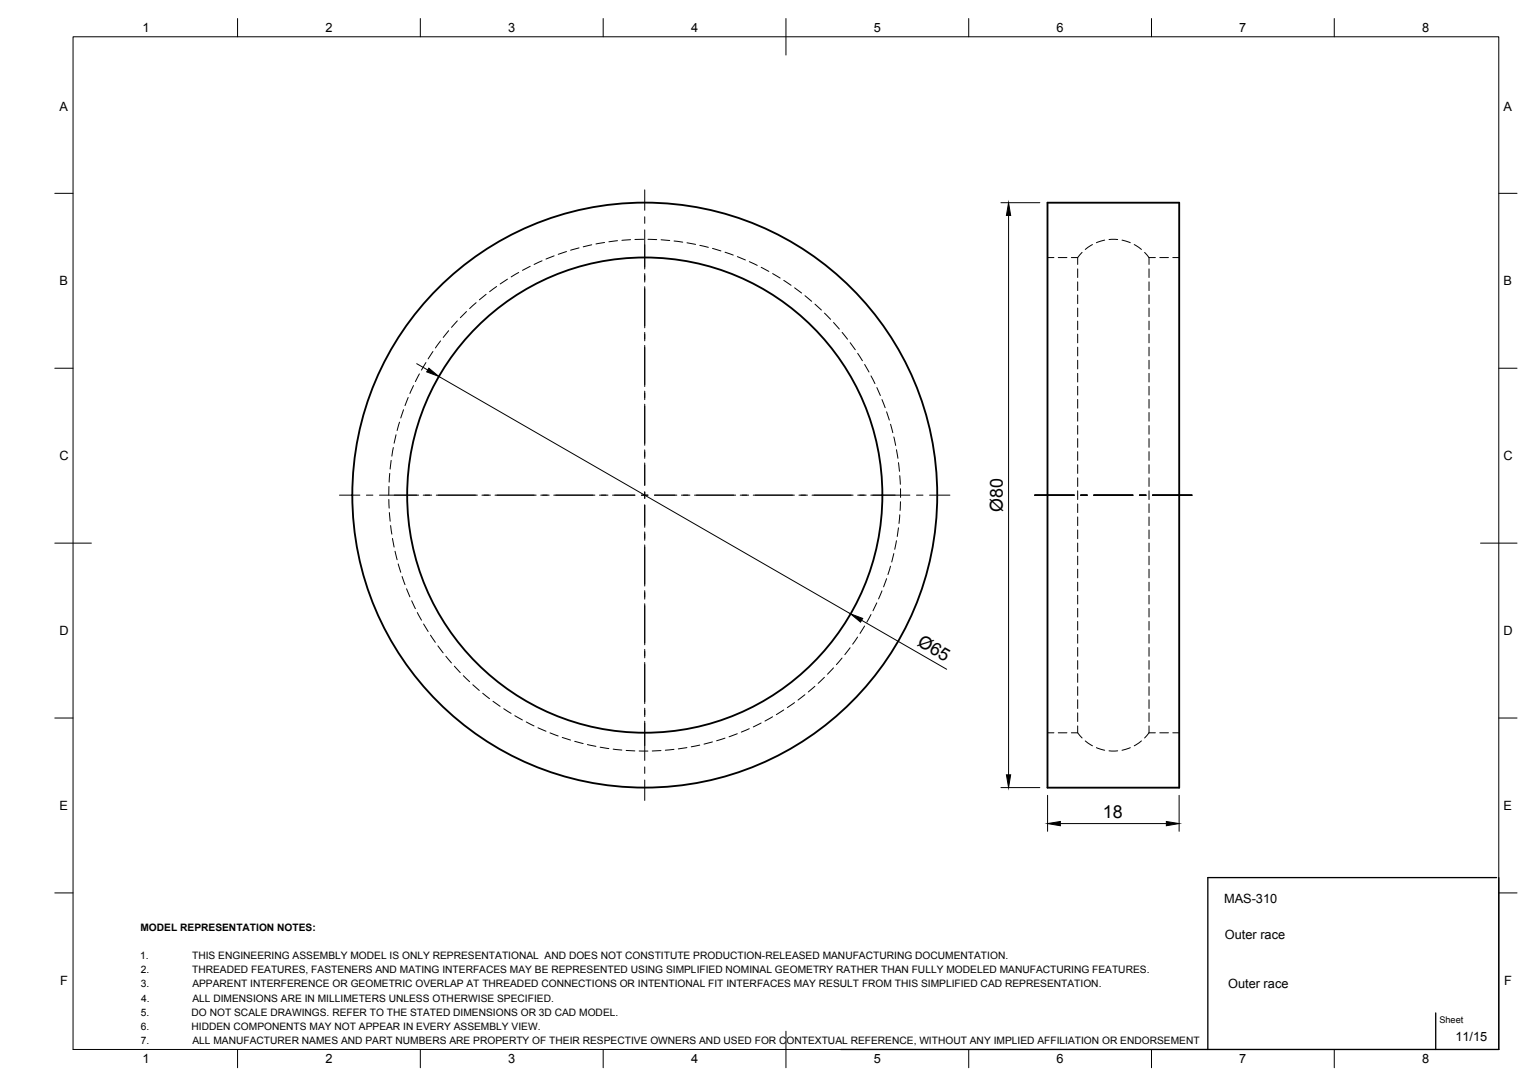
ISO-10303-21;
HEADER;
/* Generated by software containing ST-Developer
 * from STEP Tools, Inc. (www.steptools.com) 
 */

FILE_DESCRIPTION(
/* description */ ('Independent30mm screw-fed quill/spindle unit with16mm straight tool s
ocket, radial set screw, native reusable open ball bearings, retained 
inner/outer race stacks, keyed quill guide and M12x1.75 fine feed. Ext
ernal moving drive and tool not included. Ideal cage orbital links; in
dividual ball spin, force and preload not simulated. No drilling capac
ity, runout, speed, torque, load, life or machine safety rating.'),
/* implementation_level */ '2;1');

FILE_NAME(
/* name */ 'Outer race.step',
/* time_stamp */ '2026-11-08T18:59:42-08:00',
/* author */ (''),
/* organization */ (''),
/* preprocessor_version */ 'ST-DEVELOPER v20.2',
/* originating_system */ 'Autodesk Translation Framework v15.17.0.0',
/* authorisation */ '');

FILE_SCHEMA (('AUTOMOTIVE_DESIGN { 1 0 10303 214 3 1 1 }'));
ENDSEC;

DATA;
#10=MECHANICAL_DESIGN_GEOMETRIC_PRESENTATION_REPRESENTATION('',(#1605),#63898);
#237=TOROIDAL_SURFACE('',#16635,29.,6.);
#1569=SHAPE_REPRESENTATION_RELATIONSHIP('SRR','None',#64008,#1587);
#1587=ADVANCED_BREP_SHAPE_REPRESENTATION('',(#1623),#63893);
#1605=STYLED_ITEM('',(#64103),#1623);
#1623=MANIFOLD_SOLID_BREP('Body1',#15491);
#1708=FACE_BOUND('',#4335,.T.);
#1709=FACE_BOUND('',#4337,.T.);
#2338=CYLINDRICAL_SURFACE('',#16639,32.5);
#2339=CYLINDRICAL_SURFACE('',#16641,32.5);
#2340=CYLINDRICAL_SURFACE('',#16643,40.);
#2577=CIRCLE('',#16636,32.5);
#2578=CIRCLE('',#16637,6.);
#2579=CIRCLE('',#16638,32.5);
#2580=CIRCLE('',#16640,32.5);
#2581=CIRCLE('',#16642,32.5);
#2582=CIRCLE('',#16644,40.);
#2583=CIRCLE('',#16645,40.);
#3412=FACE_OUTER_BOUND('',#4330,.T.);
#3413=FACE_OUTER_BOUND('',#4331,.T.);
#3414=FACE_OUTER_BOUND('',#4332,.T.);
#3415=FACE_OUTER_BOUND('',#4333,.T.);
#3416=FACE_OUTER_BOUND('',#4334,.T.);
#3417=FACE_OUTER_BOUND('',#4336,.T.);
#4330=EDGE_LOOP('',(#14010,#14011,#14012,#14013));
#4331=EDGE_LOOP('',(#14014,#14015,#14016,#14017));
#4332=EDGE_LOOP('',(#14018,#14019,#14020,#14021));
#4333=EDGE_LOOP('',(#14022,#14023,#14024,#14025));
#4334=EDGE_LOOP('',(#14026));
#4335=EDGE_LOOP('',(#14027));
#4336=EDGE_LOOP('',(#14028));
#4337=EDGE_LOOP('',(#14029));
#5127=LINE('',#60412,#5890);
#5128=LINE('',#60415,#5891);
#5129=LINE('',#60421,#5892);
#5890=VECTOR('',#19455,32.5);
#5891=VECTOR('',#19458,32.5);
#5892=VECTOR('',#19465,40.);
#7336=VERTEX_POINT('',#60404);
#7337=VERTEX_POINT('',#60406);
#7338=VERTEX_POINT('',#60410);
#7339=VERTEX_POINT('',#60414);
#7340=VERTEX_POINT('',#60418);
#7341=VERTEX_POINT('',#60420);
#9594=EDGE_CURVE('',#7336,#7336,#2577,.T.);
#9595=EDGE_CURVE('',#7336,#7337,#2578,.T.);
#9596=EDGE_CURVE('',#7337,#7337,#2579,.T.);
#9597=EDGE_CURVE('',#7338,#7338,#2580,.T.);
#9598=EDGE_CURVE('',#7338,#7337,#5127,.T.);
#9599=EDGE_CURVE('',#7336,#7339,#5128,.T.);
#9600=EDGE_CURVE('',#7339,#7339,#2581,.T.);
#9601=EDGE_CURVE('',#7340,#7340,#2582,.T.);
#9602=EDGE_CURVE('',#7340,#7341,#5129,.T.);
#9603=EDGE_CURVE('',#7341,#7341,#2583,.T.);
#14010=ORIENTED_EDGE('',*,*,#9594,.F.);
#14011=ORIENTED_EDGE('',*,*,#9595,.T.);
#14012=ORIENTED_EDGE('',*,*,#9596,.F.);
#14013=ORIENTED_EDGE('',*,*,#9595,.F.);
#14014=ORIENTED_EDGE('',*,*,#9597,.F.);
#14015=ORIENTED_EDGE('',*,*,#9598,.T.);
#14016=ORIENTED_EDGE('',*,*,#9596,.T.);
#14017=ORIENTED_EDGE('',*,*,#9598,.F.);
#14018=ORIENTED_EDGE('',*,*,#9594,.T.);
#14019=ORIENTED_EDGE('',*,*,#9599,.T.);
#14020=ORIENTED_EDGE('',*,*,#9600,.T.);
#14021=ORIENTED_EDGE('',*,*,#9599,.F.);
#14022=ORIENTED_EDGE('',*,*,#9601,.F.);
#14023=ORIENTED_EDGE('',*,*,#9602,.T.);
#14024=ORIENTED_EDGE('',*,*,#9603,.T.);
#14025=ORIENTED_EDGE('',*,*,#9602,.F.);
#14026=ORIENTED_EDGE('',*,*,#9601,.T.);
#14027=ORIENTED_EDGE('',*,*,#9597,.T.);
#14028=ORIENTED_EDGE('',*,*,#9603,.F.);
#14029=ORIENTED_EDGE('',*,*,#9600,.F.);
#14613=PLANE('',#16646);
#14614=PLANE('',#16647);
#15392=ADVANCED_FACE('',(#3412),#237,.F.);
#15393=ADVANCED_FACE('',(#3413),#2338,.F.);
#15394=ADVANCED_FACE('',(#3414),#2339,.F.);
#15395=ADVANCED_FACE('',(#3415),#2340,.T.);
#15396=ADVANCED_FACE('',(#3416,#1708),#14613,.T.);
#15397=ADVANCED_FACE('',(#3417,#1709),#14614,.F.);
#15491=CLOSED_SHELL('',(#15392,#15393,#15394,#15395,#15396,#15397));
#16634=AXIS2_PLACEMENT_3D('',#60402,#19441,#19442);
#16635=AXIS2_PLACEMENT_3D('',#60403,#19443,#19444);
#16636=AXIS2_PLACEMENT_3D('',#60405,#19445,#19446);
#16637=AXIS2_PLACEMENT_3D('',#60407,#19447,#19448);
#16638=AXIS2_PLACEMENT_3D('',#60408,#19449,#19450);
#16639=AXIS2_PLACEMENT_3D('',#60409,#19451,#19452);
#16640=AXIS2_PLACEMENT_3D('',#60411,#19453,#19454);
#16641=AXIS2_PLACEMENT_3D('',#60413,#19456,#19457);
#16642=AXIS2_PLACEMENT_3D('',#60416,#19459,#19460);
#16643=AXIS2_PLACEMENT_3D('',#60417,#19461,#19462);
#16644=AXIS2_PLACEMENT_3D('',#60419,#19463,#19464);
#16645=AXIS2_PLACEMENT_3D('',#60422,#19466,#19467);
#16646=AXIS2_PLACEMENT_3D('',#60423,#19468,#19469);
#16647=AXIS2_PLACEMENT_3D('',#60424,#19470,#19471);
#19441=DIRECTION('axis',(0.,0.,1.));
#19442=DIRECTION('refdir',(1.,0.,0.));
#19443=DIRECTION('center_axis',(0.,0.,1.));
#19444=DIRECTION('ref_axis',(1.,0.,0.));
#19445=DIRECTION('center_axis',(0.,0.,1.));
#19446=DIRECTION('ref_axis',(1.,0.,0.));
#19447=DIRECTION('center_axis',(-1.22464679914735E-16,1.,0.));
#19448=DIRECTION('ref_axis',(-1.,-1.22464679914735E-16,0.));
#19449=DIRECTION('center_axis',(0.,0.,-1.));
#19450=DIRECTION('ref_axis',(1.,0.,0.));
#19451=DIRECTION('center_axis',(0.,0.,1.));
#19452=DIRECTION('ref_axis',(1.,0.,0.));
#19453=DIRECTION('center_axis',(0.,0.,-1.));
#19454=DIRECTION('ref_axis',(1.,0.,0.));
#19455=DIRECTION('',(0.,0.,-1.));
#19456=DIRECTION('center_axis',(0.,0.,1.));
#19457=DIRECTION('ref_axis',(1.,0.,0.));
#19458=DIRECTION('',(0.,0.,-1.));
#19459=DIRECTION('center_axis',(0.,0.,-1.));
#19460=DIRECTION('ref_axis',(1.,0.,0.));
#19461=DIRECTION('center_axis',(0.,0.,1.));
#19462=DIRECTION('ref_axis',(1.,0.,0.));
#19463=DIRECTION('center_axis',(0.,0.,1.));
#19464=DIRECTION('ref_axis',(1.,0.,0.));
#19465=DIRECTION('',(0.,0.,-1.));
#19466=DIRECTION('center_axis',(0.,0.,1.));
#19467=DIRECTION('ref_axis',(1.,0.,0.));
#19468=DIRECTION('center_axis',(0.,0.,1.));
#19469=DIRECTION('ref_axis',(1.,0.,0.));
#19470=DIRECTION('center_axis',(0.,0.,1.));
#19471=DIRECTION('ref_axis',(1.,0.,0.));
#60402=CARTESIAN_POINT('',(0.,0.,0.));
#60403=CARTESIAN_POINT('Origin',(0.,0.,0.));
#60404=CARTESIAN_POINT('',(-32.5,-3.9801020972289E-15,-4.87339717240448));
#60405=CARTESIAN_POINT('Origin',(0.,0.,-4.87339717240448));
#60406=CARTESIAN_POINT('',(-32.5,3.9801020972289E-15,4.87339717240448));
#60407=CARTESIAN_POINT('Origin',(-29.,-3.55147571752732E-15,0.));
#60408=CARTESIAN_POINT('Origin',(0.,0.,4.87339717240448));
#60409=CARTESIAN_POINT('Origin',(0.,0.,-9.));
#60410=CARTESIAN_POINT('',(-32.5,-3.9801020972289E-15,9.));
#60411=CARTESIAN_POINT('Origin',(0.,0.,9.));
#60412=CARTESIAN_POINT('',(-32.5,-3.9801020972289E-15,-9.));
#60413=CARTESIAN_POINT('Origin',(0.,0.,-9.));
#60414=CARTESIAN_POINT('',(-32.5,-3.9801020972289E-15,-9.));
#60415=CARTESIAN_POINT('',(-32.5,-3.9801020972289E-15,-9.));
#60416=CARTESIAN_POINT('Origin',(0.,0.,-9.));
#60417=CARTESIAN_POINT('Origin',(0.,0.,-9.));
#60418=CARTESIAN_POINT('',(-40.,-4.89858719658941E-15,9.));
#60419=CARTESIAN_POINT('Origin',(0.,0.,9.));
#60420=CARTESIAN_POINT('',(-40.,-4.89858719658941E-15,-9.));
#60421=CARTESIAN_POINT('',(-40.,-4.89858719658941E-15,-9.));
#60422=CARTESIAN_POINT('Origin',(0.,0.,-9.));
#60423=CARTESIAN_POINT('Origin',(0.,0.,9.));
#60424=CARTESIAN_POINT('Origin',(0.,0.,-9.));
#63873=UNCERTAINTY_MEASURE_WITH_UNIT(LENGTH_MEASURE(0.01),#63899,
'DISTANCE_ACCURACY_VALUE',
'Maximum model space distance between geometric entities at asserted c
onnectivities');
#63878=UNCERTAINTY_MEASURE_WITH_UNIT(LENGTH_MEASURE(0.01),#63899,
'DISTANCE_ACCURACY_VALUE',
'Maximum model space distance between geometric entities at asserted c
onnectivities');
#63893=(
GEOMETRIC_REPRESENTATION_CONTEXT(3)
GLOBAL_UNCERTAINTY_ASSIGNED_CONTEXT((#63873))
GLOBAL_UNIT_ASSIGNED_CONTEXT((#63899,#63901,#63902))
REPRESENTATION_CONTEXT('','3D')
);
#63898=(
GEOMETRIC_REPRESENTATION_CONTEXT(3)
GLOBAL_UNCERTAINTY_ASSIGNED_CONTEXT((#63878))
GLOBAL_UNIT_ASSIGNED_CONTEXT((#63899,#63901,#63902))
REPRESENTATION_CONTEXT('','3D')
);
#63899=(
LENGTH_UNIT()
NAMED_UNIT(*)
SI_UNIT(.MILLI.,.METRE.)
);
#63901=(
NAMED_UNIT(*)
PLANE_ANGLE_UNIT()
SI_UNIT($,.RADIAN.)
);
#63902=(
NAMED_UNIT(*)
SI_UNIT($,.STERADIAN.)
SOLID_ANGLE_UNIT()
);
#63917=SHAPE_DEFINITION_REPRESENTATION(#63936,#64008);
#63936=PRODUCT_DEFINITION_SHAPE('',$,#64028);
#64008=SHAPE_REPRESENTATION('',(#16634),#63893);
#64013=PRODUCT_DEFINITION_CONTEXT('part definition',#64072,'design');
#64028=PRODUCT_DEFINITION('Outer race','Outer race',#64047,#64013);
#64047=PRODUCT_DEFINITION_FORMATION('',$,#64088);
#64072=APPLICATION_CONTEXT(
'Core Data for Automotive Mechanical Design Process');
#64073=PRODUCT_CONTEXT('part definition',#64072,'mechanical');
#64088=PRODUCT('Outer race','Outer race',$,(#64073));
#64103=PRESENTATION_STYLE_ASSIGNMENT((#64116));
#64116=SURFACE_STYLE_USAGE(.BOTH.,#64129);
#64129=SURFACE_SIDE_STYLE('',(#64142));
#64142=SURFACE_STYLE_FILL_AREA(#64155);
#64155=FILL_AREA_STYLE('Outer race gray',(#64168));
#64168=FILL_AREA_STYLE_COLOUR('Outer race gray',#64181);
#64181=COLOUR_RGB('Outer race gray',0.407843137254902,0.447058823529412,
0.498039215686275);
ENDSEC;
END-ISO-10303-21;
